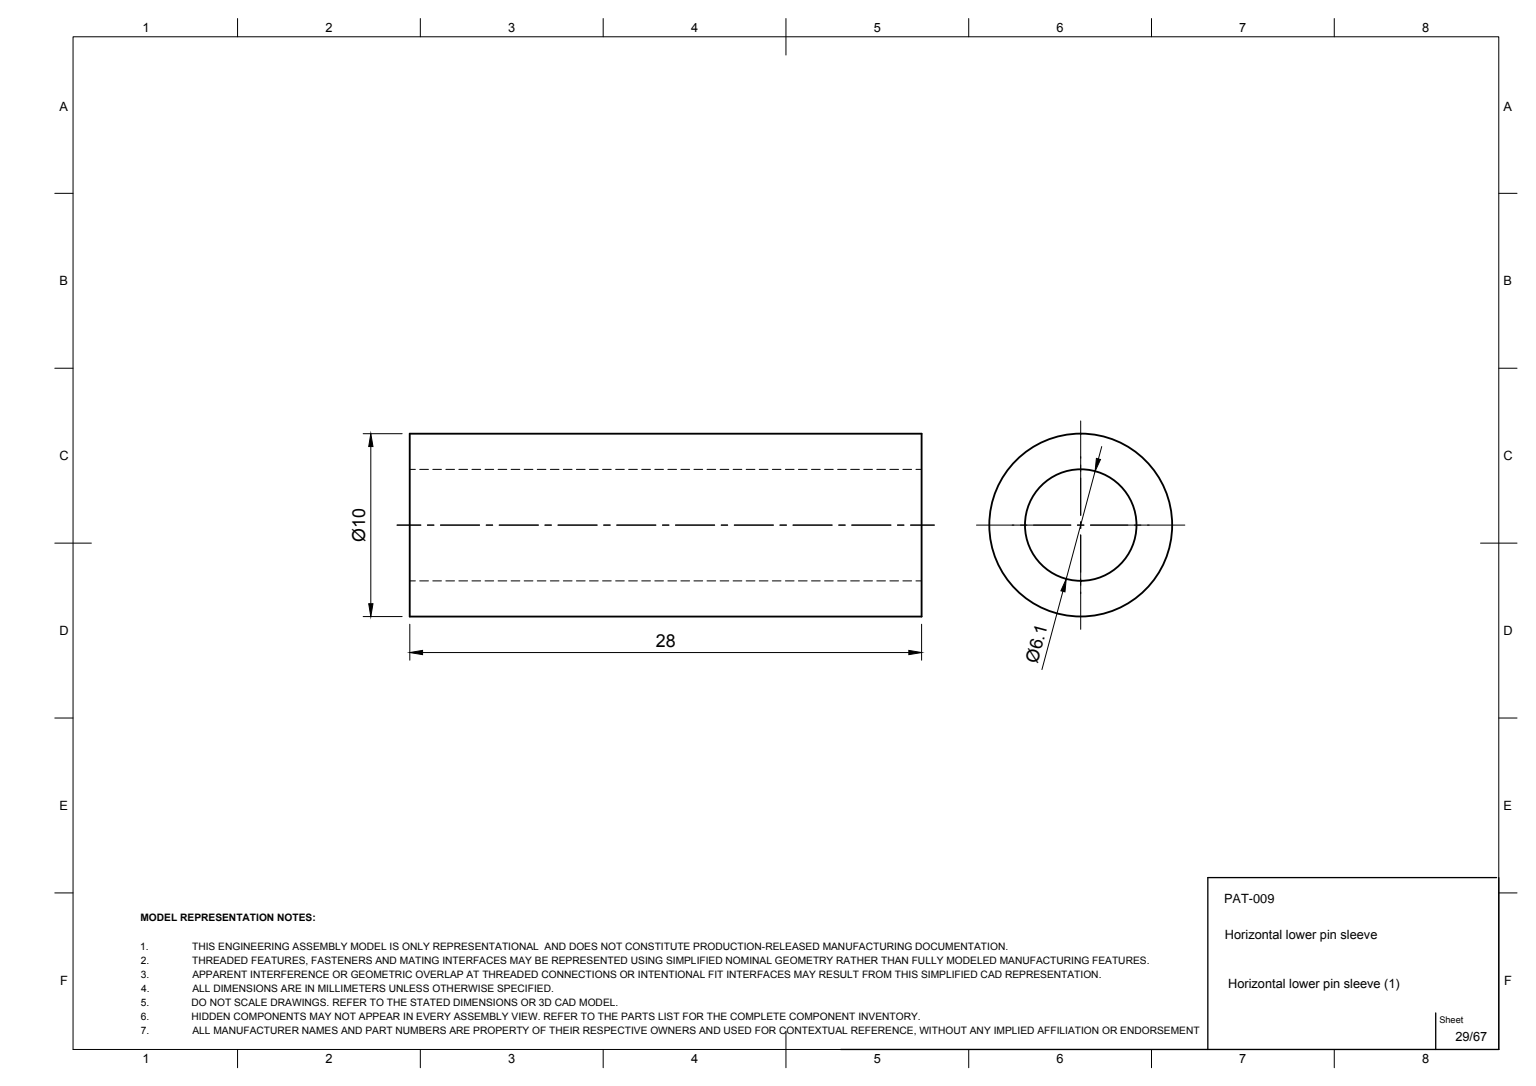
ISO-10303-21;
HEADER;
/* Generated by software containing ST-Developer
 * from STEP Tools, Inc. (www.steptools.com) 
 */

FILE_DESCRIPTION(
/* description */ ('Bell-crank linkage with push rods'),
/* implementation_level */ '2;1');

FILE_NAME(
/* name */ 'Horizontal lower pin sleeve.step',
/* time_stamp */ '2026-10-28T03:25:15-07:00',
/* author */ (''),
/* organization */ (''),
/* preprocessor_version */ 'ST-DEVELOPER v20.2',
/* originating_system */ 'Autodesk Translation Framework v15.17.0.0',
/* authorisation */ '');

FILE_SCHEMA (('AUTOMOTIVE_DESIGN { 1 0 10303 214 3 1 1 }'));
ENDSEC;

DATA;
#10=MECHANICAL_DESIGN_GEOMETRIC_PRESENTATION_REPRESENTATION('',(#634),#16678);
#518=SHAPE_REPRESENTATION_RELATIONSHIP('SRR','None',#16936,#572);
#572=ADVANCED_BREP_SHAPE_REPRESENTATION('',(#695),#16641);
#634=STYLED_ITEM('',(#17291),#695);
#695=MANIFOLD_SOLID_BREP('Body1',#8825);
#841=FACE_BOUND('',#2164,.T.);
#842=FACE_BOUND('',#2166,.T.);
#1106=PLANE('',#10050);
#1107=PLANE('',#10051);
#1523=FACE_OUTER_BOUND('',#2161,.T.);
#1524=FACE_OUTER_BOUND('',#2162,.T.);
#1525=FACE_OUTER_BOUND('',#2163,.T.);
#1526=FACE_OUTER_BOUND('',#2165,.T.);
#2161=EDGE_LOOP('',(#7129,#7130,#7131,#7132));
#2162=EDGE_LOOP('',(#7133,#7134,#7135,#7136));
#2163=EDGE_LOOP('',(#7137));
#2164=EDGE_LOOP('',(#7138));
#2165=EDGE_LOOP('',(#7139));
#2166=EDGE_LOOP('',(#7140));
#2820=LINE('',#15398,#3369);
#2821=LINE('',#15404,#3370);
#3369=VECTOR('',#12102,0.305);
#3370=VECTOR('',#12109,0.5);
#3912=CIRCLE('',#10045,0.305);
#3913=CIRCLE('',#10046,0.305);
#3914=CIRCLE('',#10048,0.5);
#3915=CIRCLE('',#10049,0.5);
#4523=VERTEX_POINT('',#15395);
#4524=VERTEX_POINT('',#15397);
#4525=VERTEX_POINT('',#15401);
#4526=VERTEX_POINT('',#15403);
#5442=EDGE_CURVE('',#4523,#4523,#3912,.T.);
#5443=EDGE_CURVE('',#4523,#4524,#2820,.T.);
#5444=EDGE_CURVE('',#4524,#4524,#3913,.T.);
#5445=EDGE_CURVE('',#4525,#4525,#3914,.T.);
#5446=EDGE_CURVE('',#4525,#4526,#2821,.T.);
#5447=EDGE_CURVE('',#4526,#4526,#3915,.T.);
#7129=ORIENTED_EDGE('',*,*,#5442,.F.);
#7130=ORIENTED_EDGE('',*,*,#5443,.T.);
#7131=ORIENTED_EDGE('',*,*,#5444,.T.);
#7132=ORIENTED_EDGE('',*,*,#5443,.F.);
#7133=ORIENTED_EDGE('',*,*,#5445,.F.);
#7134=ORIENTED_EDGE('',*,*,#5446,.T.);
#7135=ORIENTED_EDGE('',*,*,#5447,.T.);
#7136=ORIENTED_EDGE('',*,*,#5446,.F.);
#7137=ORIENTED_EDGE('',*,*,#5445,.T.);
#7138=ORIENTED_EDGE('',*,*,#5442,.T.);
#7139=ORIENTED_EDGE('',*,*,#5447,.F.);
#7140=ORIENTED_EDGE('',*,*,#5444,.F.);
#8175=CYLINDRICAL_SURFACE('',#10044,0.305);
#8176=CYLINDRICAL_SURFACE('',#10047,0.5);
#8548=ADVANCED_FACE('',(#1523),#8175,.F.);
#8549=ADVANCED_FACE('',(#1524),#8176,.T.);
#8550=ADVANCED_FACE('',(#1525,#841),#1106,.T.);
#8551=ADVANCED_FACE('',(#1526,#842),#1107,.F.);
#8825=CLOSED_SHELL('',(#8548,#8549,#8550,#8551));
#10043=AXIS2_PLACEMENT_3D('',#15393,#12096,#12097);
#10044=AXIS2_PLACEMENT_3D('',#15394,#12098,#12099);
#10045=AXIS2_PLACEMENT_3D('',#15396,#12100,#12101);
#10046=AXIS2_PLACEMENT_3D('',#15399,#12103,#12104);
#10047=AXIS2_PLACEMENT_3D('',#15400,#12105,#12106);
#10048=AXIS2_PLACEMENT_3D('',#15402,#12107,#12108);
#10049=AXIS2_PLACEMENT_3D('',#15405,#12110,#12111);
#10050=AXIS2_PLACEMENT_3D('',#15406,#12112,#12113);
#10051=AXIS2_PLACEMENT_3D('',#15407,#12114,#12115);
#12096=DIRECTION('axis',(0.,0.,1.));
#12097=DIRECTION('refdir',(1.,0.,0.));
#12098=DIRECTION('center_axis',(0.,0.,1.));
#12099=DIRECTION('ref_axis',(1.,0.,0.));
#12100=DIRECTION('center_axis',(0.,0.,-1.));
#12101=DIRECTION('ref_axis',(1.,0.,0.));
#12102=DIRECTION('',(0.,0.,-1.));
#12103=DIRECTION('center_axis',(0.,0.,-1.));
#12104=DIRECTION('ref_axis',(1.,0.,0.));
#12105=DIRECTION('center_axis',(0.,0.,1.));
#12106=DIRECTION('ref_axis',(1.,0.,0.));
#12107=DIRECTION('center_axis',(0.,0.,1.));
#12108=DIRECTION('ref_axis',(1.,0.,0.));
#12109=DIRECTION('',(0.,0.,-1.));
#12110=DIRECTION('center_axis',(0.,0.,1.));
#12111=DIRECTION('ref_axis',(1.,0.,0.));
#12112=DIRECTION('center_axis',(0.,0.,1.));
#12113=DIRECTION('ref_axis',(1.,0.,0.));
#12114=DIRECTION('center_axis',(0.,0.,1.));
#12115=DIRECTION('ref_axis',(1.,0.,0.));
#15393=CARTESIAN_POINT('',(0.,0.,0.));
#15394=CARTESIAN_POINT('Origin',(0.,2.,6.));
#15395=CARTESIAN_POINT('',(-0.305,2.,8.8));
#15396=CARTESIAN_POINT('Origin',(0.,2.,8.8));
#15397=CARTESIAN_POINT('',(-0.305,2.,6.));
#15398=CARTESIAN_POINT('',(-0.305,2.,6.));
#15399=CARTESIAN_POINT('Origin',(0.,2.,6.));
#15400=CARTESIAN_POINT('Origin',(0.,2.,6.));
#15401=CARTESIAN_POINT('',(-0.5,2.,8.8));
#15402=CARTESIAN_POINT('Origin',(0.,2.,8.8));
#15403=CARTESIAN_POINT('',(-0.5,2.,6.));
#15404=CARTESIAN_POINT('',(-0.5,2.,6.));
#15405=CARTESIAN_POINT('Origin',(0.,2.,6.));
#15406=CARTESIAN_POINT('Origin',(0.,2.,8.8));
#15407=CARTESIAN_POINT('Origin',(0.,2.,6.));
#16577=UNCERTAINTY_MEASURE_WITH_UNIT(LENGTH_MEASURE(0.001),#16679,
'DISTANCE_ACCURACY_VALUE',
'Maximum model space distance between geometric entities at asserted c
onnectivities');
#16614=UNCERTAINTY_MEASURE_WITH_UNIT(LENGTH_MEASURE(0.001),#16679,
'DISTANCE_ACCURACY_VALUE',
'Maximum model space distance between geometric entities at asserted c
onnectivities');
#16641=(
GEOMETRIC_REPRESENTATION_CONTEXT(3)
GLOBAL_UNCERTAINTY_ASSIGNED_CONTEXT((#16577))
GLOBAL_UNIT_ASSIGNED_CONTEXT((#16679,#16681,#16682))
REPRESENTATION_CONTEXT('','3D')
);
#16678=(
GEOMETRIC_REPRESENTATION_CONTEXT(3)
GLOBAL_UNCERTAINTY_ASSIGNED_CONTEXT((#16614))
GLOBAL_UNIT_ASSIGNED_CONTEXT((#16679,#16681,#16682))
REPRESENTATION_CONTEXT('','3D')
);
#16679=(
LENGTH_UNIT()
NAMED_UNIT(*)
SI_UNIT(.CENTI.,.METRE.)
);
#16681=(
NAMED_UNIT(*)
PLANE_ANGLE_UNIT()
SI_UNIT($,.RADIAN.)
);
#16682=(
NAMED_UNIT(*)
SI_UNIT($,.STERADIAN.)
SOLID_ANGLE_UNIT()
);
#16709=SHAPE_DEFINITION_REPRESENTATION(#16777,#16936);
#16777=PRODUCT_DEFINITION_SHAPE('',$,#17000);
#16936=SHAPE_REPRESENTATION('',(#10043),#16641);
#16973=PRODUCT_DEFINITION_CONTEXT('part definition',#17164,'design');
#17000=PRODUCT_DEFINITION('Horizontal lower pin sleeve',
'Horizontal lower pin sleeve',#17063,#16973);
#17063=PRODUCT_DEFINITION_FORMATION('',$,#17192);
#17164=APPLICATION_CONTEXT(
'Core Data for Automotive Mechanical Design Process');
#17165=PRODUCT_CONTEXT('part definition',#17164,'mechanical');
#17192=PRODUCT('Horizontal lower pin sleeve',
'Horizontal lower pin sleeve','Horizontal lower pin sleeve',(#17165));
#17285=COLOUR_RGB('Grey',0.48,0.52,0.57);
#17286=FILL_AREA_STYLE_COLOUR('',#17285);
#17287=FILL_AREA_STYLE('',(#17286));
#17288=SURFACE_STYLE_FILL_AREA(#17287);
#17289=SURFACE_SIDE_STYLE('',(#17288));
#17290=SURFACE_STYLE_USAGE(.BOTH.,#17289);
#17291=PRESENTATION_STYLE_ASSIGNMENT((#17290));
ENDSEC;
END-ISO-10303-21;
